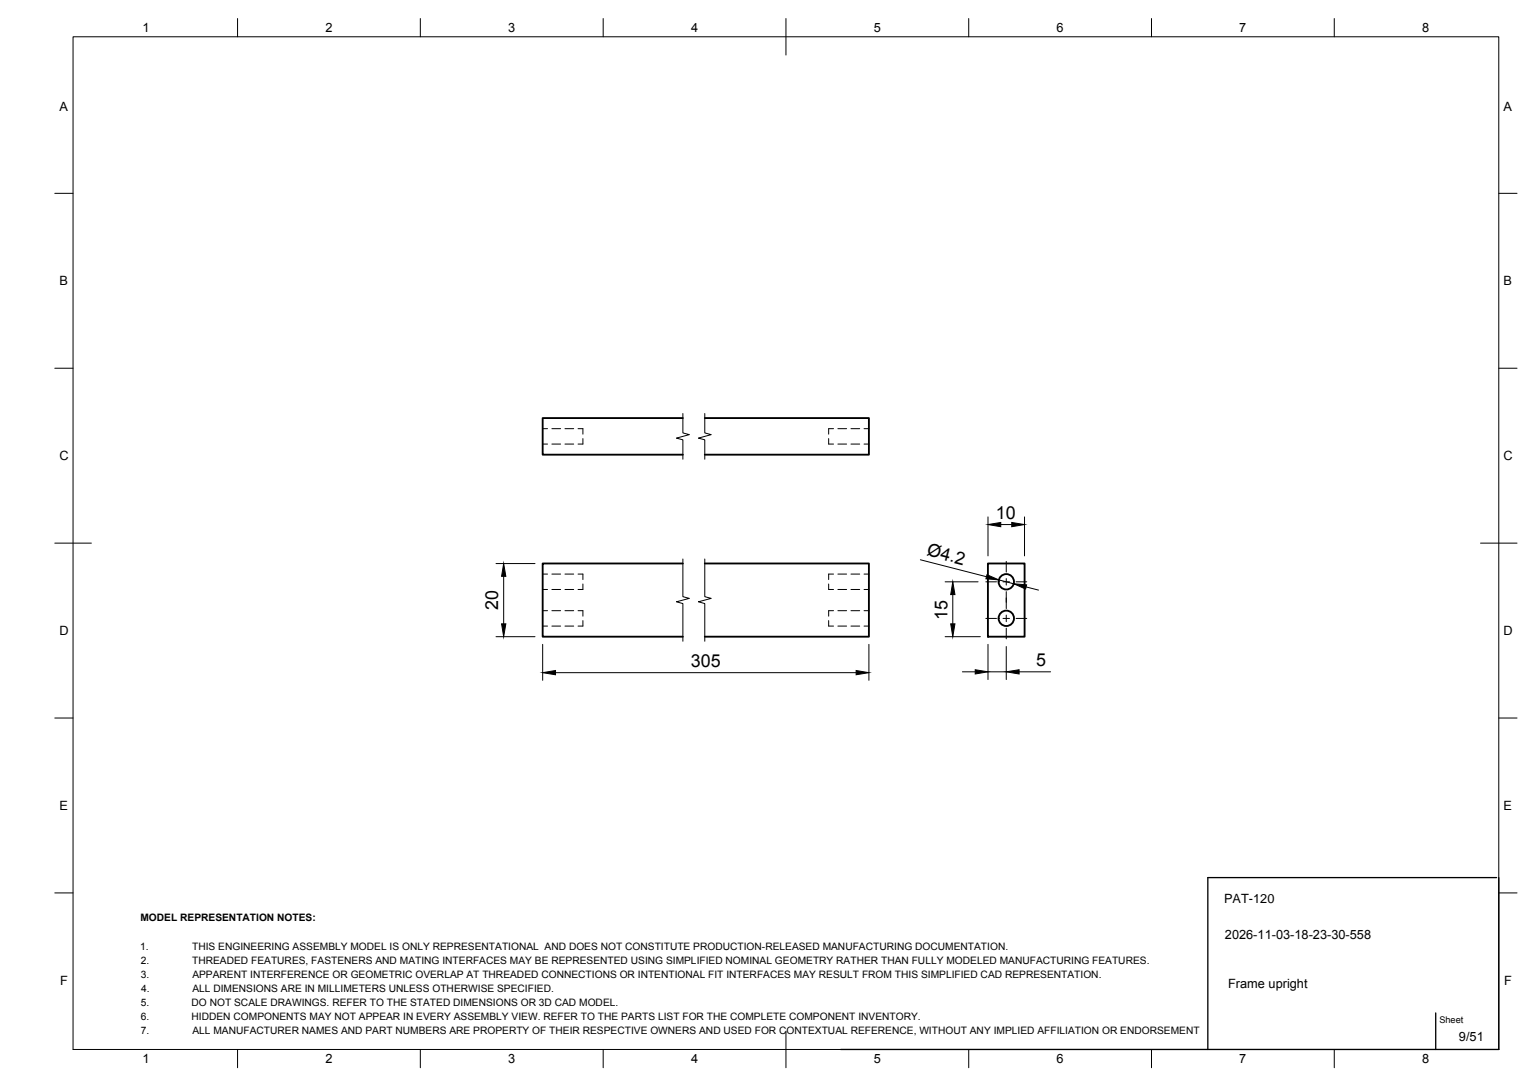
ISO-10303-21;
HEADER;
/* Generated by software containing ST-Developer
 * from STEP Tools, Inc. (www.steptools.com) 
 */

FILE_DESCRIPTION(
/* description */ ('Vibration shaker table dummy'),
/* implementation_level */ '2;1');

FILE_NAME(
/* name */ 'Frame upright.step',
/* time_stamp */ '2026-10-27T10:55:14-07:00',
/* author */ (''),
/* organization */ (''),
/* preprocessor_version */ 'ST-DEVELOPER v20.2',
/* originating_system */ 'Autodesk Translation Framework v15.17.0.0',
/* authorisation */ '');

FILE_SCHEMA (('AUTOMOTIVE_DESIGN { 1 0 10303 214 3 1 1 }'));
ENDSEC;

DATA;
#10=MECHANICAL_DESIGN_GEOMETRIC_PRESENTATION_REPRESENTATION('',(#690),#22394);
#598=SHAPE_REPRESENTATION_RELATIONSHIP('SRR','None',#22644,#644);
#644=ADVANCED_BREP_SHAPE_REPRESENTATION('',(#736),#22350);
#690=STYLED_ITEM('',(#22940),#736);
#736=MANIFOLD_SOLID_BREP('Body1',#9208);
#855=FACE_BOUND('',#1996,.T.);
#856=FACE_BOUND('',#1997,.T.);
#857=FACE_BOUND('',#1999,.T.);
#858=FACE_BOUND('',#2000,.T.);
#1084=PLANE('',#9914);
#1085=PLANE('',#9918);
#1086=PLANE('',#9922);
#1087=PLANE('',#9926);
#1088=PLANE('',#9927);
#1089=PLANE('',#9928);
#1090=PLANE('',#9929);
#1091=PLANE('',#9930);
#1092=PLANE('',#9931);
#1093=PLANE('',#9932);
#1405=FACE_OUTER_BOUND('',#1983,.T.);
#1406=FACE_OUTER_BOUND('',#1984,.T.);
#1407=FACE_OUTER_BOUND('',#1985,.T.);
#1408=FACE_OUTER_BOUND('',#1986,.T.);
#1409=FACE_OUTER_BOUND('',#1987,.T.);
#1410=FACE_OUTER_BOUND('',#1988,.T.);
#1411=FACE_OUTER_BOUND('',#1989,.T.);
#1412=FACE_OUTER_BOUND('',#1990,.T.);
#1413=FACE_OUTER_BOUND('',#1991,.T.);
#1414=FACE_OUTER_BOUND('',#1992,.T.);
#1415=FACE_OUTER_BOUND('',#1993,.T.);
#1416=FACE_OUTER_BOUND('',#1994,.T.);
#1417=FACE_OUTER_BOUND('',#1995,.T.);
#1418=FACE_OUTER_BOUND('',#1998,.T.);
#1983=EDGE_LOOP('',(#6582,#6583,#6584,#6585));
#1984=EDGE_LOOP('',(#6586));
#1985=EDGE_LOOP('',(#6587,#6588,#6589,#6590));
#1986=EDGE_LOOP('',(#6591));
#1987=EDGE_LOOP('',(#6592,#6593,#6594,#6595));
#1988=EDGE_LOOP('',(#6596));
#1989=EDGE_LOOP('',(#6597,#6598,#6599,#6600));
#1990=EDGE_LOOP('',(#6601));
#1991=EDGE_LOOP('',(#6602,#6603,#6604,#6605));
#1992=EDGE_LOOP('',(#6606,#6607,#6608,#6609));
#1993=EDGE_LOOP('',(#6610,#6611,#6612,#6613));
#1994=EDGE_LOOP('',(#6614,#6615,#6616,#6617));
#1995=EDGE_LOOP('',(#6618,#6619,#6620,#6621));
#1996=EDGE_LOOP('',(#6622));
#1997=EDGE_LOOP('',(#6623));
#1998=EDGE_LOOP('',(#6624,#6625,#6626,#6627));
#1999=EDGE_LOOP('',(#6628));
#2000=EDGE_LOOP('',(#6629));
#2710=LINE('',#14304,#3329);
#2711=LINE('',#14311,#3330);
#2712=LINE('',#14318,#3331);
#2713=LINE('',#14325,#3332);
#2714=LINE('',#14331,#3333);
#2715=LINE('',#14333,#3334);
#2716=LINE('',#14335,#3335);
#2717=LINE('',#14336,#3336);
#2718=LINE('',#14339,#3337);
#2719=LINE('',#14341,#3338);
#2720=LINE('',#14342,#3339);
#2721=LINE('',#14345,#3340);
#2722=LINE('',#14347,#3341);
#2723=LINE('',#14348,#3342);
#2724=LINE('',#14350,#3343);
#2725=LINE('',#14351,#3344);
#3329=VECTOR('',#11344,0.210000000000001);
#3330=VECTOR('',#11353,0.210000000000001);
#3331=VECTOR('',#11362,0.210000000000001);
#3332=VECTOR('',#11371,0.210000000000001);
#3333=VECTOR('',#11378,1.);
#3334=VECTOR('',#11379,1.);
#3335=VECTOR('',#11380,1.);
#3336=VECTOR('',#11381,1.);
#3337=VECTOR('',#11384,1.);
#3338=VECTOR('',#11385,1.);
#3339=VECTOR('',#11386,1.);
#3340=VECTOR('',#11389,1.);
#3341=VECTOR('',#11390,1.);
#3342=VECTOR('',#11391,1.);
#3343=VECTOR('',#11394,1.);
#3344=VECTOR('',#11395,1.);
#3940=CIRCLE('',#9912,0.210000000000001);
#3941=CIRCLE('',#9913,0.210000000000001);
#3942=CIRCLE('',#9916,0.210000000000001);
#3943=CIRCLE('',#9917,0.210000000000001);
#3944=CIRCLE('',#9920,0.210000000000001);
#3945=CIRCLE('',#9921,0.210000000000001);
#3946=CIRCLE('',#9924,0.210000000000001);
#3947=CIRCLE('',#9925,0.210000000000001);
#4479=VERTEX_POINT('',#14301);
#4480=VERTEX_POINT('',#14303);
#4481=VERTEX_POINT('',#14308);
#4482=VERTEX_POINT('',#14310);
#4483=VERTEX_POINT('',#14315);
#4484=VERTEX_POINT('',#14317);
#4485=VERTEX_POINT('',#14322);
#4486=VERTEX_POINT('',#14324);
#4487=VERTEX_POINT('',#14329);
#4488=VERTEX_POINT('',#14330);
#4489=VERTEX_POINT('',#14332);
#4490=VERTEX_POINT('',#14334);
#4491=VERTEX_POINT('',#14338);
#4492=VERTEX_POINT('',#14340);
#4493=VERTEX_POINT('',#14344);
#4494=VERTEX_POINT('',#14346);
#5284=EDGE_CURVE('',#4479,#4479,#3940,.T.);
#5285=EDGE_CURVE('',#4479,#4480,#2710,.T.);
#5286=EDGE_CURVE('',#4480,#4480,#3941,.T.);
#5287=EDGE_CURVE('',#4481,#4481,#3942,.T.);
#5288=EDGE_CURVE('',#4481,#4482,#2711,.T.);
#5289=EDGE_CURVE('',#4482,#4482,#3943,.T.);
#5290=EDGE_CURVE('',#4483,#4483,#3944,.T.);
#5291=EDGE_CURVE('',#4483,#4484,#2712,.T.);
#5292=EDGE_CURVE('',#4484,#4484,#3945,.T.);
#5293=EDGE_CURVE('',#4485,#4485,#3946,.T.);
#5294=EDGE_CURVE('',#4485,#4486,#2713,.T.);
#5295=EDGE_CURVE('',#4486,#4486,#3947,.T.);
#5296=EDGE_CURVE('',#4487,#4488,#2714,.T.);
#5297=EDGE_CURVE('',#4488,#4489,#2715,.T.);
#5298=EDGE_CURVE('',#4490,#4489,#2716,.T.);
#5299=EDGE_CURVE('',#4487,#4490,#2717,.T.);
#5300=EDGE_CURVE('',#4491,#4487,#2718,.T.);
#5301=EDGE_CURVE('',#4492,#4490,#2719,.T.);
#5302=EDGE_CURVE('',#4491,#4492,#2720,.T.);
#5303=EDGE_CURVE('',#4493,#4491,#2721,.T.);
#5304=EDGE_CURVE('',#4494,#4492,#2722,.T.);
#5305=EDGE_CURVE('',#4493,#4494,#2723,.T.);
#5306=EDGE_CURVE('',#4488,#4493,#2724,.T.);
#5307=EDGE_CURVE('',#4489,#4494,#2725,.T.);
#6582=ORIENTED_EDGE('',*,*,#5284,.F.);
#6583=ORIENTED_EDGE('',*,*,#5285,.T.);
#6584=ORIENTED_EDGE('',*,*,#5286,.F.);
#6585=ORIENTED_EDGE('',*,*,#5285,.F.);
#6586=ORIENTED_EDGE('',*,*,#5284,.T.);
#6587=ORIENTED_EDGE('',*,*,#5287,.F.);
#6588=ORIENTED_EDGE('',*,*,#5288,.T.);
#6589=ORIENTED_EDGE('',*,*,#5289,.F.);
#6590=ORIENTED_EDGE('',*,*,#5288,.F.);
#6591=ORIENTED_EDGE('',*,*,#5287,.T.);
#6592=ORIENTED_EDGE('',*,*,#5290,.F.);
#6593=ORIENTED_EDGE('',*,*,#5291,.T.);
#6594=ORIENTED_EDGE('',*,*,#5292,.T.);
#6595=ORIENTED_EDGE('',*,*,#5291,.F.);
#6596=ORIENTED_EDGE('',*,*,#5292,.F.);
#6597=ORIENTED_EDGE('',*,*,#5293,.F.);
#6598=ORIENTED_EDGE('',*,*,#5294,.T.);
#6599=ORIENTED_EDGE('',*,*,#5295,.T.);
#6600=ORIENTED_EDGE('',*,*,#5294,.F.);
#6601=ORIENTED_EDGE('',*,*,#5295,.F.);
#6602=ORIENTED_EDGE('',*,*,#5296,.T.);
#6603=ORIENTED_EDGE('',*,*,#5297,.T.);
#6604=ORIENTED_EDGE('',*,*,#5298,.F.);
#6605=ORIENTED_EDGE('',*,*,#5299,.F.);
#6606=ORIENTED_EDGE('',*,*,#5300,.T.);
#6607=ORIENTED_EDGE('',*,*,#5299,.T.);
#6608=ORIENTED_EDGE('',*,*,#5301,.F.);
#6609=ORIENTED_EDGE('',*,*,#5302,.F.);
#6610=ORIENTED_EDGE('',*,*,#5303,.T.);
#6611=ORIENTED_EDGE('',*,*,#5302,.T.);
#6612=ORIENTED_EDGE('',*,*,#5304,.F.);
#6613=ORIENTED_EDGE('',*,*,#5305,.F.);
#6614=ORIENTED_EDGE('',*,*,#5306,.T.);
#6615=ORIENTED_EDGE('',*,*,#5305,.T.);
#6616=ORIENTED_EDGE('',*,*,#5307,.F.);
#6617=ORIENTED_EDGE('',*,*,#5297,.F.);
#6618=ORIENTED_EDGE('',*,*,#5307,.T.);
#6619=ORIENTED_EDGE('',*,*,#5304,.T.);
#6620=ORIENTED_EDGE('',*,*,#5301,.T.);
#6621=ORIENTED_EDGE('',*,*,#5298,.T.);
#6622=ORIENTED_EDGE('',*,*,#5286,.T.);
#6623=ORIENTED_EDGE('',*,*,#5289,.T.);
#6624=ORIENTED_EDGE('',*,*,#5306,.F.);
#6625=ORIENTED_EDGE('',*,*,#5296,.F.);
#6626=ORIENTED_EDGE('',*,*,#5300,.F.);
#6627=ORIENTED_EDGE('',*,*,#5303,.F.);
#6628=ORIENTED_EDGE('',*,*,#5290,.T.);
#6629=ORIENTED_EDGE('',*,*,#5293,.T.);
#8546=CYLINDRICAL_SURFACE('',#9911,0.210000000000001);
#8547=CYLINDRICAL_SURFACE('',#9915,0.210000000000001);
#8548=CYLINDRICAL_SURFACE('',#9919,0.210000000000001);
#8549=CYLINDRICAL_SURFACE('',#9923,0.210000000000001);
#8770=ADVANCED_FACE('',(#1405),#8546,.F.);
#8771=ADVANCED_FACE('',(#1406),#1084,.T.);
#8772=ADVANCED_FACE('',(#1407),#8547,.F.);
#8773=ADVANCED_FACE('',(#1408),#1085,.T.);
#8774=ADVANCED_FACE('',(#1409),#8548,.F.);
#8775=ADVANCED_FACE('',(#1410),#1086,.F.);
#8776=ADVANCED_FACE('',(#1411),#8549,.F.);
#8777=ADVANCED_FACE('',(#1412),#1087,.F.);
#8778=ADVANCED_FACE('',(#1413),#1088,.T.);
#8779=ADVANCED_FACE('',(#1414),#1089,.T.);
#8780=ADVANCED_FACE('',(#1415),#1090,.T.);
#8781=ADVANCED_FACE('',(#1416),#1091,.T.);
#8782=ADVANCED_FACE('',(#1417,#855,#856),#1092,.T.);
#8783=ADVANCED_FACE('',(#1418,#857,#858),#1093,.F.);
#9208=CLOSED_SHELL('',(#8770,#8771,#8772,#8773,#8774,#8775,#8776,#8777,
#8778,#8779,#8780,#8781,#8782,#8783));
#9910=AXIS2_PLACEMENT_3D('',#14299,#11338,#11339);
#9911=AXIS2_PLACEMENT_3D('',#14300,#11340,#11341);
#9912=AXIS2_PLACEMENT_3D('',#14302,#11342,#11343);
#9913=AXIS2_PLACEMENT_3D('',#14305,#11345,#11346);
#9914=AXIS2_PLACEMENT_3D('',#14306,#11347,#11348);
#9915=AXIS2_PLACEMENT_3D('',#14307,#11349,#11350);
#9916=AXIS2_PLACEMENT_3D('',#14309,#11351,#11352);
#9917=AXIS2_PLACEMENT_3D('',#14312,#11354,#11355);
#9918=AXIS2_PLACEMENT_3D('',#14313,#11356,#11357);
#9919=AXIS2_PLACEMENT_3D('',#14314,#11358,#11359);
#9920=AXIS2_PLACEMENT_3D('',#14316,#11360,#11361);
#9921=AXIS2_PLACEMENT_3D('',#14319,#11363,#11364);
#9922=AXIS2_PLACEMENT_3D('',#14320,#11365,#11366);
#9923=AXIS2_PLACEMENT_3D('',#14321,#11367,#11368);
#9924=AXIS2_PLACEMENT_3D('',#14323,#11369,#11370);
#9925=AXIS2_PLACEMENT_3D('',#14326,#11372,#11373);
#9926=AXIS2_PLACEMENT_3D('',#14327,#11374,#11375);
#9927=AXIS2_PLACEMENT_3D('',#14328,#11376,#11377);
#9928=AXIS2_PLACEMENT_3D('',#14337,#11382,#11383);
#9929=AXIS2_PLACEMENT_3D('',#14343,#11387,#11388);
#9930=AXIS2_PLACEMENT_3D('',#14349,#11392,#11393);
#9931=AXIS2_PLACEMENT_3D('',#14352,#11396,#11397);
#9932=AXIS2_PLACEMENT_3D('',#14353,#11398,#11399);
#11338=DIRECTION('axis',(0.,0.,1.));
#11339=DIRECTION('refdir',(1.,0.,0.));
#11340=DIRECTION('center_axis',(0.,0.,1.));
#11341=DIRECTION('ref_axis',(1.,0.,0.));
#11342=DIRECTION('center_axis',(0.,0.,1.));
#11343=DIRECTION('ref_axis',(1.,0.,0.));
#11344=DIRECTION('',(0.,0.,1.));
#11345=DIRECTION('center_axis',(0.,0.,-1.));
#11346=DIRECTION('ref_axis',(1.,0.,0.));
#11347=DIRECTION('center_axis',(0.,0.,1.));
#11348=DIRECTION('ref_axis',(1.,0.,0.));
#11349=DIRECTION('center_axis',(0.,0.,1.));
#11350=DIRECTION('ref_axis',(1.,0.,0.));
#11351=DIRECTION('center_axis',(0.,0.,1.));
#11352=DIRECTION('ref_axis',(1.,0.,0.));
#11353=DIRECTION('',(0.,0.,1.));
#11354=DIRECTION('center_axis',(0.,0.,-1.));
#11355=DIRECTION('ref_axis',(1.,0.,0.));
#11356=DIRECTION('center_axis',(0.,0.,1.));
#11357=DIRECTION('ref_axis',(1.,0.,0.));
#11358=DIRECTION('center_axis',(0.,0.,1.));
#11359=DIRECTION('ref_axis',(1.,0.,0.));
#11360=DIRECTION('center_axis',(0.,0.,1.));
#11361=DIRECTION('ref_axis',(1.,0.,0.));
#11362=DIRECTION('',(0.,0.,1.));
#11363=DIRECTION('center_axis',(0.,0.,1.));
#11364=DIRECTION('ref_axis',(1.,0.,0.));
#11365=DIRECTION('center_axis',(0.,0.,1.));
#11366=DIRECTION('ref_axis',(1.,0.,0.));
#11367=DIRECTION('center_axis',(0.,0.,1.));
#11368=DIRECTION('ref_axis',(1.,0.,0.));
#11369=DIRECTION('center_axis',(0.,0.,1.));
#11370=DIRECTION('ref_axis',(1.,0.,0.));
#11371=DIRECTION('',(0.,0.,1.));
#11372=DIRECTION('center_axis',(0.,0.,1.));
#11373=DIRECTION('ref_axis',(1.,0.,0.));
#11374=DIRECTION('center_axis',(0.,0.,1.));
#11375=DIRECTION('ref_axis',(1.,0.,0.));
#11376=DIRECTION('center_axis',(0.,1.,0.));
#11377=DIRECTION('ref_axis',(-1.,0.,0.));
#11378=DIRECTION('',(-1.,0.,0.));
#11379=DIRECTION('',(0.,0.,1.));
#11380=DIRECTION('',(-1.,0.,0.));
#11381=DIRECTION('',(0.,0.,1.));
#11382=DIRECTION('center_axis',(1.,0.,0.));
#11383=DIRECTION('ref_axis',(0.,1.,0.));
#11384=DIRECTION('',(0.,1.,0.));
#11385=DIRECTION('',(0.,1.,0.));
#11386=DIRECTION('',(0.,0.,1.));
#11387=DIRECTION('center_axis',(0.,-1.,0.));
#11388=DIRECTION('ref_axis',(1.,0.,0.));
#11389=DIRECTION('',(1.,0.,0.));
#11390=DIRECTION('',(1.,0.,0.));
#11391=DIRECTION('',(0.,0.,1.));
#11392=DIRECTION('center_axis',(-1.,0.,0.));
#11393=DIRECTION('ref_axis',(0.,-1.,0.));
#11394=DIRECTION('',(0.,-1.,0.));
#11395=DIRECTION('',(0.,-1.,0.));
#11396=DIRECTION('center_axis',(0.,0.,1.));
#11397=DIRECTION('ref_axis',(1.,0.,0.));
#11398=DIRECTION('center_axis',(0.,0.,1.));
#11399=DIRECTION('ref_axis',(1.,0.,0.));
#14299=CARTESIAN_POINT('',(0.,0.,0.));
#14300=CARTESIAN_POINT('Origin',(-9.5,10.,29.4));
#14301=CARTESIAN_POINT('',(-9.71,10.,29.4));
#14302=CARTESIAN_POINT('Origin',(-9.5,10.,29.4));
#14303=CARTESIAN_POINT('',(-9.71,10.,30.5));
#14304=CARTESIAN_POINT('',(-9.71,10.,29.4));
#14305=CARTESIAN_POINT('Origin',(-9.5,10.,30.5));
#14306=CARTESIAN_POINT('Origin',(-9.5,10.,29.4));
#14307=CARTESIAN_POINT('Origin',(-9.5,11.,29.4));
#14308=CARTESIAN_POINT('',(-9.71,11.,29.4));
#14309=CARTESIAN_POINT('Origin',(-9.5,11.,29.4));
#14310=CARTESIAN_POINT('',(-9.71,11.,30.5));
#14311=CARTESIAN_POINT('',(-9.71,11.,29.4));
#14312=CARTESIAN_POINT('Origin',(-9.5,11.,30.5));
#14313=CARTESIAN_POINT('Origin',(-9.5,11.,29.4));
#14314=CARTESIAN_POINT('Origin',(-9.5,10.,-0.1));
#14315=CARTESIAN_POINT('',(-9.71,10.,0.));
#14316=CARTESIAN_POINT('Origin',(-9.5,10.,0.));
#14317=CARTESIAN_POINT('',(-9.71,10.,1.1));
#14318=CARTESIAN_POINT('',(-9.71,10.,-0.1));
#14319=CARTESIAN_POINT('Origin',(-9.5,10.,1.1));
#14320=CARTESIAN_POINT('Origin',(-9.5,10.,1.1));
#14321=CARTESIAN_POINT('Origin',(-9.5,11.,-0.1));
#14322=CARTESIAN_POINT('',(-9.71,11.,0.));
#14323=CARTESIAN_POINT('Origin',(-9.5,11.,0.));
#14324=CARTESIAN_POINT('',(-9.71,11.,1.1));
#14325=CARTESIAN_POINT('',(-9.71,11.,-0.1));
#14326=CARTESIAN_POINT('Origin',(-9.5,11.,1.1));
#14327=CARTESIAN_POINT('Origin',(-9.5,11.,1.1));
#14328=CARTESIAN_POINT('Origin',(-9.,11.5,0.));
#14329=CARTESIAN_POINT('',(-9.,11.5,0.));
#14330=CARTESIAN_POINT('',(-10.,11.5,0.));
#14331=CARTESIAN_POINT('',(-9.,11.5,0.));
#14332=CARTESIAN_POINT('',(-10.,11.5,30.5));
#14333=CARTESIAN_POINT('',(-10.,11.5,0.));
#14334=CARTESIAN_POINT('',(-9.,11.5,30.5));
#14335=CARTESIAN_POINT('',(-9.,11.5,30.5));
#14336=CARTESIAN_POINT('',(-9.,11.5,0.));
#14337=CARTESIAN_POINT('Origin',(-9.,9.5,0.));
#14338=CARTESIAN_POINT('',(-9.,9.5,0.));
#14339=CARTESIAN_POINT('',(-9.,9.5,0.));
#14340=CARTESIAN_POINT('',(-9.,9.5,30.5));
#14341=CARTESIAN_POINT('',(-9.,9.5,30.5));
#14342=CARTESIAN_POINT('',(-9.,9.5,0.));
#14343=CARTESIAN_POINT('Origin',(-10.,9.5,0.));
#14344=CARTESIAN_POINT('',(-10.,9.5,0.));
#14345=CARTESIAN_POINT('',(-10.,9.5,0.));
#14346=CARTESIAN_POINT('',(-10.,9.5,30.5));
#14347=CARTESIAN_POINT('',(-10.,9.5,30.5));
#14348=CARTESIAN_POINT('',(-10.,9.5,0.));
#14349=CARTESIAN_POINT('Origin',(-10.,11.5,0.));
#14350=CARTESIAN_POINT('',(-10.,11.5,0.));
#14351=CARTESIAN_POINT('',(-10.,11.5,30.5));
#14352=CARTESIAN_POINT('Origin',(-9.5,10.5,30.5));
#14353=CARTESIAN_POINT('Origin',(-9.5,10.5,0.));
#22299=UNCERTAINTY_MEASURE_WITH_UNIT(LENGTH_MEASURE(0.001),#22395,
'DISTANCE_ACCURACY_VALUE',
'Maximum model space distance between geometric entities at asserted c
onnectivities');
#22343=UNCERTAINTY_MEASURE_WITH_UNIT(LENGTH_MEASURE(0.001),#22395,
'DISTANCE_ACCURACY_VALUE',
'Maximum model space distance between geometric entities at asserted c
onnectivities');
#22350=(
GEOMETRIC_REPRESENTATION_CONTEXT(3)
GLOBAL_UNCERTAINTY_ASSIGNED_CONTEXT((#22299))
GLOBAL_UNIT_ASSIGNED_CONTEXT((#22395,#22397,#22398))
REPRESENTATION_CONTEXT('','3D')
);
#22394=(
GEOMETRIC_REPRESENTATION_CONTEXT(3)
GLOBAL_UNCERTAINTY_ASSIGNED_CONTEXT((#22343))
GLOBAL_UNIT_ASSIGNED_CONTEXT((#22395,#22397,#22398))
REPRESENTATION_CONTEXT('','3D')
);
#22395=(
LENGTH_UNIT()
NAMED_UNIT(*)
SI_UNIT(.CENTI.,.METRE.)
);
#22397=(
NAMED_UNIT(*)
PLANE_ANGLE_UNIT()
SI_UNIT($,.RADIAN.)
);
#22398=(
NAMED_UNIT(*)
SI_UNIT($,.STERADIAN.)
SOLID_ANGLE_UNIT()
);
#22405=SHAPE_DEFINITION_REPRESENTATION(#22455,#22644);
#22455=PRODUCT_DEFINITION_SHAPE('',$,#22695);
#22644=SHAPE_REPRESENTATION('',(#9910),#22350);
#22688=PRODUCT_DEFINITION_CONTEXT('part definition',#22840,'design');
#22695=PRODUCT_DEFINITION('Frame upright','Frame upright',#22745,#22688);
#22745=PRODUCT_DEFINITION_FORMATION('',$,#22848);
#22840=APPLICATION_CONTEXT(
'Core Data for Automotive Mechanical Design Process');
#22841=PRODUCT_CONTEXT('part definition',#22840,'mechanical');
#22848=PRODUCT('Frame upright','Frame upright','Frame upright',(#22841));
#22934=COLOUR_RGB('Dark Blue',0.08,0.2,0.34);
#22935=FILL_AREA_STYLE_COLOUR('',#22934);
#22936=FILL_AREA_STYLE('',(#22935));
#22937=SURFACE_STYLE_FILL_AREA(#22936);
#22938=SURFACE_SIDE_STYLE('',(#22937));
#22939=SURFACE_STYLE_USAGE(.BOTH.,#22938);
#22940=PRESENTATION_STYLE_ASSIGNMENT((#22939));
ENDSEC;
END-ISO-10303-21;
